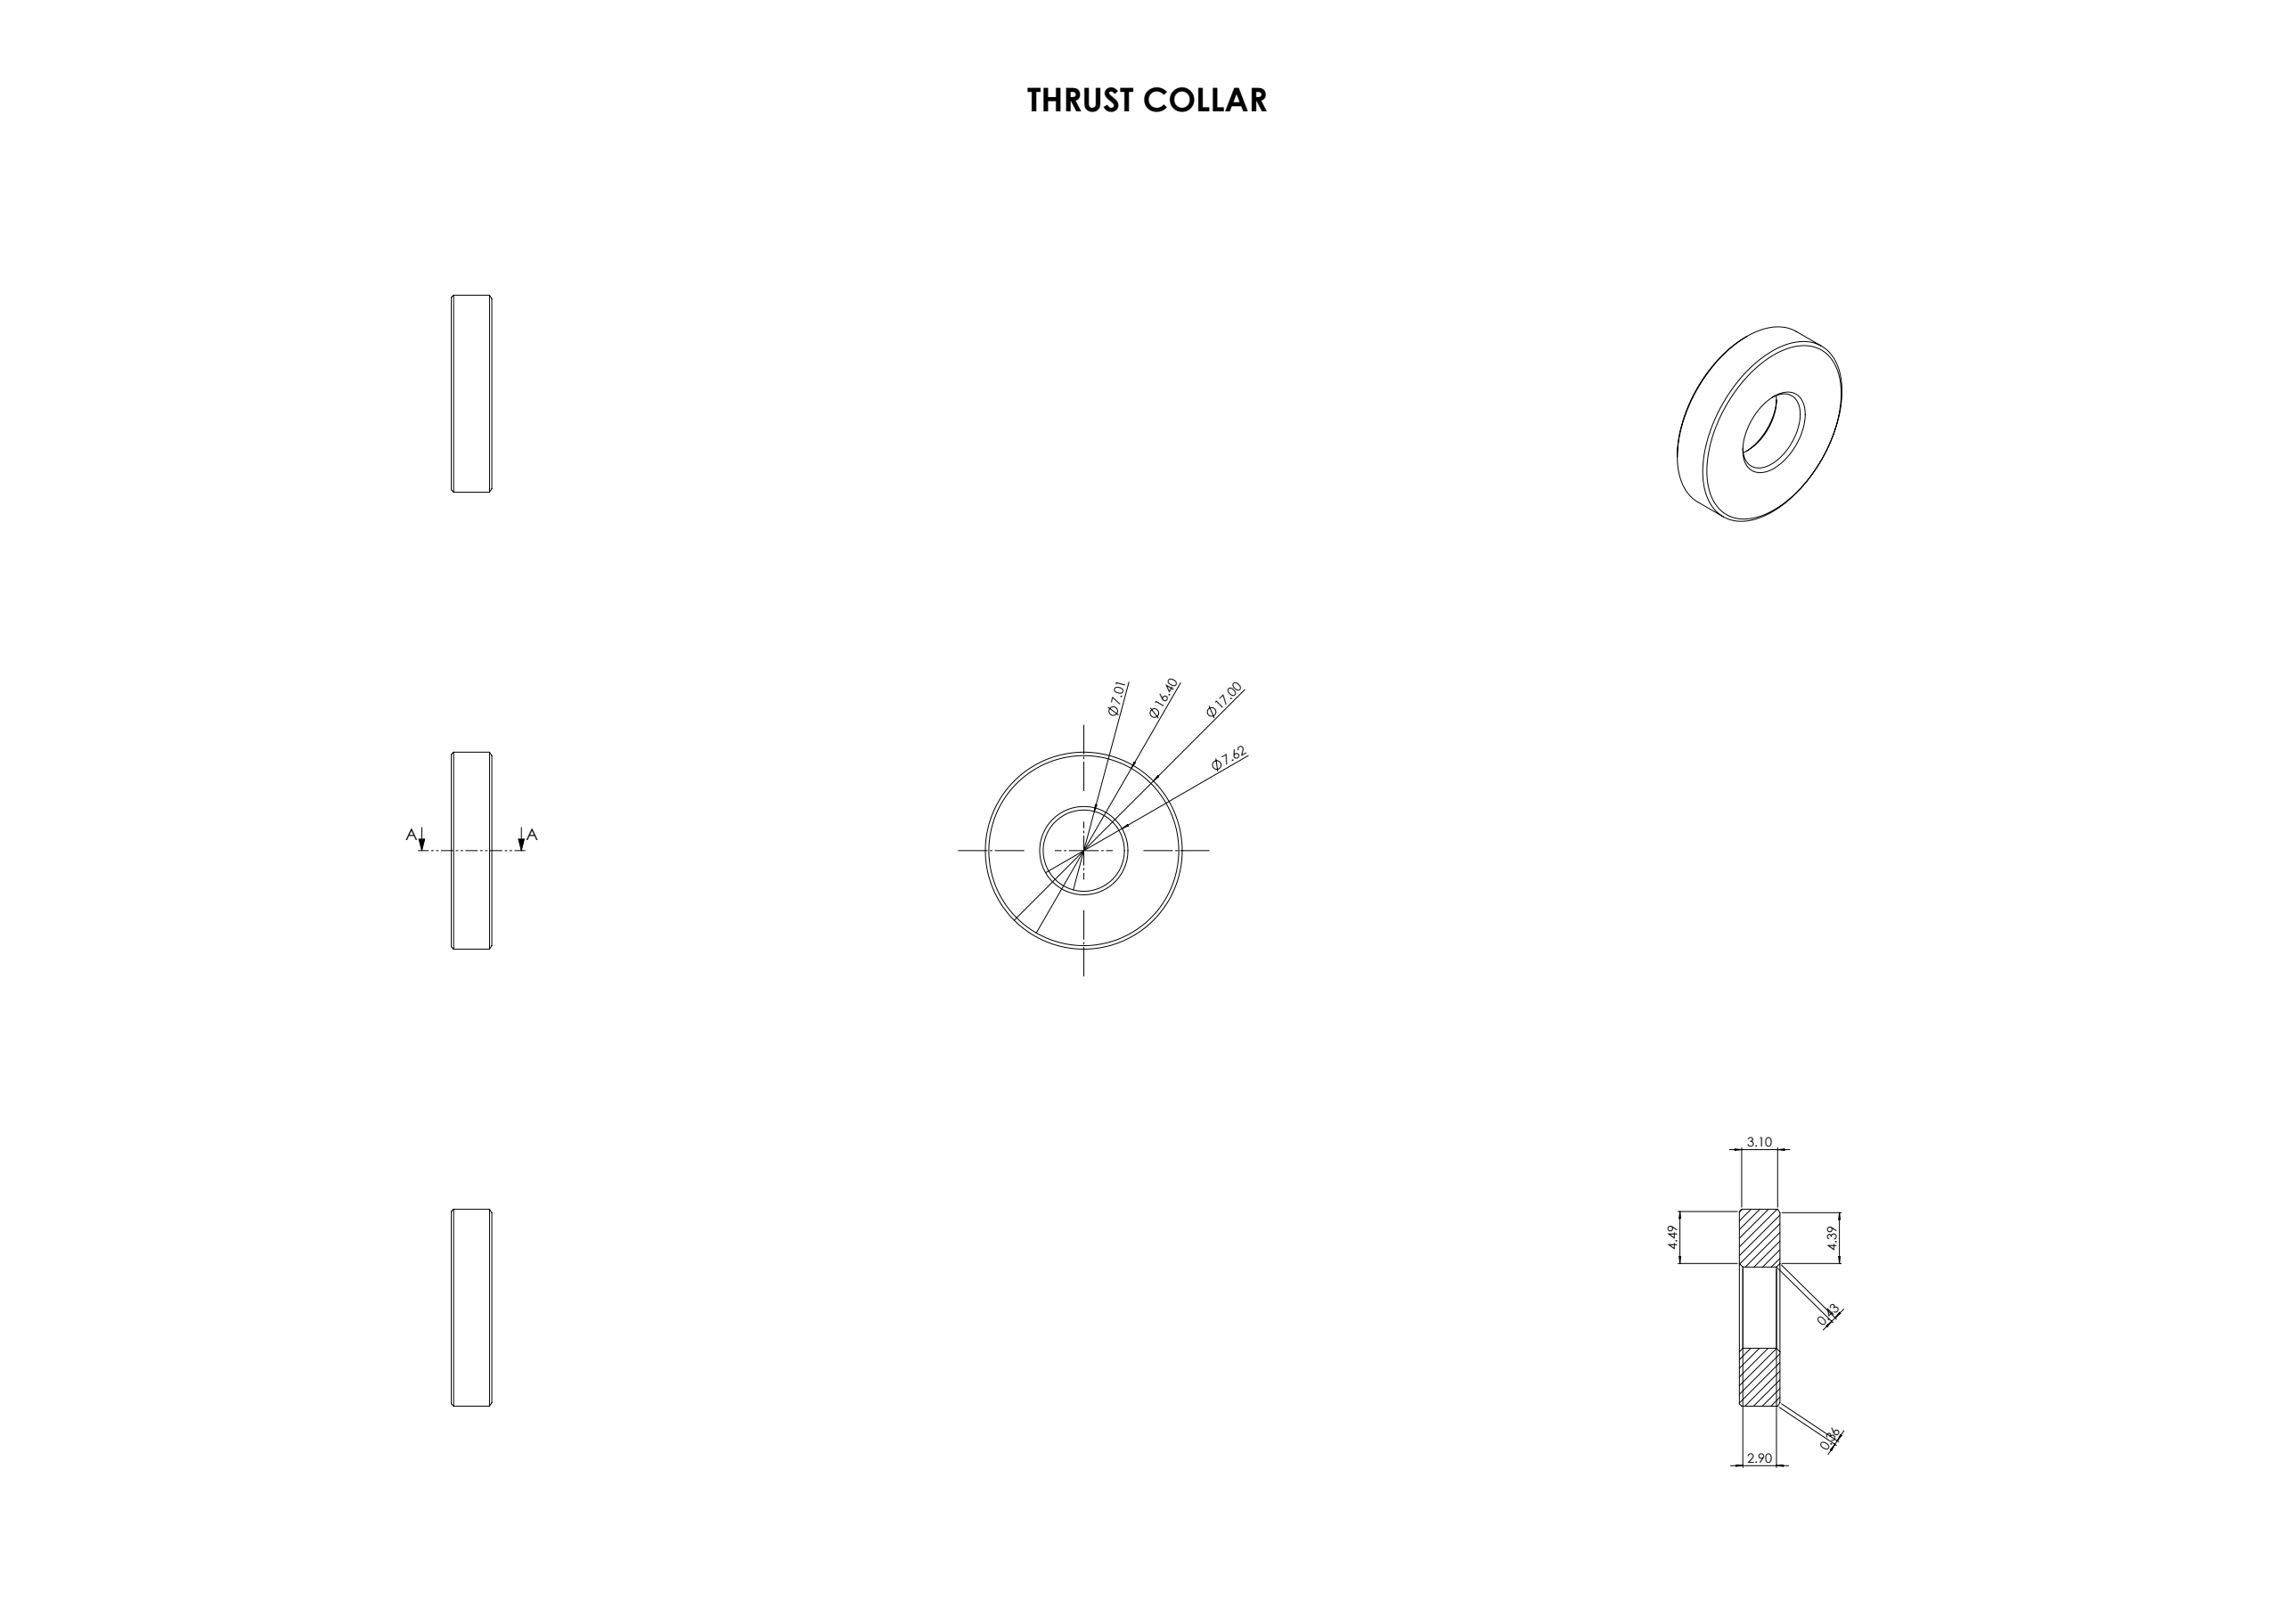
ISO-10303-21;
HEADER;
/* Generated by software containing ST-Developer
 * from STEP Tools, Inc. (www.steptools.com) 
 */

FILE_DESCRIPTION(
/* description */ (''),
/* implementation_level */ '2;1');

FILE_NAME(
/* name */ '05_Thrust_Collar.step',
/* time_stamp */ '2026-10-25T01:10:36-07:00',
/* author */ (''),
/* organization */ (''),
/* preprocessor_version */ 'ST-DEVELOPER v20.2',
/* originating_system */ 'Autodesk Translation Framework v15.15.0.0',
/* authorisation */ '');

FILE_SCHEMA (('AUTOMOTIVE_DESIGN { 1 0 10303 214 3 1 1 }'));
ENDSEC;

DATA;
#10=MECHANICAL_DESIGN_GEOMETRIC_PRESENTATION_REPRESENTATION('',(#1297),#60365);
#69=SHAPE_REPRESENTATION_RELATIONSHIP('SRR','None',#60409,#79);
#79=ADVANCED_BREP_SHAPE_REPRESENTATION('',(#89),#60357);
#89=MANIFOLD_SOLID_BREP('Body1',#18299);
#206=FACE_BOUND('',#2619,.T.);
#207=FACE_BOUND('',#2624,.T.);
#401=PLANE('',#18929);
#402=PLANE('',#18937);
#902=CONICAL_SURFACE('',#18922,8.4,0.785398163397446);
#903=CONICAL_SURFACE('',#18927,8.35,0.982793723247329);
#904=CONICAL_SURFACE('',#18931,3.6575,0.7936624380571);
#905=CONICAL_SURFACE('',#18935,3.6575,0.7936624380571);
#1297=STYLED_ITEM('',(#60541),#89);
#1642=FACE_OUTER_BOUND('',#2615,.T.);
#1643=FACE_OUTER_BOUND('',#2616,.T.);
#1644=FACE_OUTER_BOUND('',#2617,.T.);
#1645=FACE_OUTER_BOUND('',#2618,.T.);
#1646=FACE_OUTER_BOUND('',#2620,.T.);
#1647=FACE_OUTER_BOUND('',#2621,.T.);
#1648=FACE_OUTER_BOUND('',#2622,.T.);
#1649=FACE_OUTER_BOUND('',#2623,.T.);
#2615=EDGE_LOOP('',(#13723,#13724,#13725,#13726));
#2616=EDGE_LOOP('',(#13727,#13728,#13729,#13730));
#2617=EDGE_LOOP('',(#13731,#13732,#13733,#13734));
#2618=EDGE_LOOP('',(#13735));
#2619=EDGE_LOOP('',(#13736));
#2620=EDGE_LOOP('',(#13737,#13738,#13739,#13740));
#2621=EDGE_LOOP('',(#13741,#13742,#13743,#13744));
#2622=EDGE_LOOP('',(#13745,#13746,#13747,#13748));
#2623=EDGE_LOOP('',(#13749));
#2624=EDGE_LOOP('',(#13750));
#3509=CIRCLE('',#18923,8.5);
#3510=CIRCLE('',#18924,8.3);
#3511=CIRCLE('',#18926,8.5);
#3512=CIRCLE('',#18928,8.2);
#3513=CIRCLE('',#18930,3.81);
#3514=CIRCLE('',#18932,3.505);
#3515=CIRCLE('',#18934,3.505);
#3516=CIRCLE('',#18936,3.81);
#4780=LINE('',#43732,#6192);
#4781=LINE('',#43737,#6193);
#4782=LINE('',#43741,#6194);
#4783=LINE('',#43747,#6195);
#4784=LINE('',#43751,#6196);
#4785=LINE('',#43755,#6197);
#6192=VECTOR('',#20970,8.4);
#6193=VECTOR('',#20977,8.5);
#6194=VECTOR('',#20982,8.35);
#6195=VECTOR('',#20989,3.6575);
#6196=VECTOR('',#20994,3.505);
#6197=VECTOR('',#20999,3.6575);
#7954=VERTEX_POINT('',#43729);
#7955=VERTEX_POINT('',#43731);
#7956=VERTEX_POINT('',#43735);
#7957=VERTEX_POINT('',#43739);
#7958=VERTEX_POINT('',#43743);
#7959=VERTEX_POINT('',#43746);
#7960=VERTEX_POINT('',#43750);
#7961=VERTEX_POINT('',#43754);
#10069=EDGE_CURVE('',#7954,#7954,#3509,.T.);
#10070=EDGE_CURVE('',#7954,#7955,#4780,.T.);
#10071=EDGE_CURVE('',#7955,#7955,#3510,.T.);
#10072=EDGE_CURVE('',#7956,#7956,#3511,.T.);
#10073=EDGE_CURVE('',#7956,#7954,#4781,.T.);
#10074=EDGE_CURVE('',#7957,#7957,#3512,.T.);
#10075=EDGE_CURVE('',#7957,#7956,#4782,.T.);
#10076=EDGE_CURVE('',#7958,#7958,#3513,.T.);
#10077=EDGE_CURVE('',#7958,#7959,#4783,.T.);
#10078=EDGE_CURVE('',#7959,#7959,#3514,.T.);
#10079=EDGE_CURVE('',#7959,#7960,#4784,.T.);
#10080=EDGE_CURVE('',#7960,#7960,#3515,.T.);
#10081=EDGE_CURVE('',#7960,#7961,#4785,.T.);
#10082=EDGE_CURVE('',#7961,#7961,#3516,.T.);
#13723=ORIENTED_EDGE('',*,*,#10069,.F.);
#13724=ORIENTED_EDGE('',*,*,#10070,.T.);
#13725=ORIENTED_EDGE('',*,*,#10071,.T.);
#13726=ORIENTED_EDGE('',*,*,#10070,.F.);
#13727=ORIENTED_EDGE('',*,*,#10072,.F.);
#13728=ORIENTED_EDGE('',*,*,#10073,.T.);
#13729=ORIENTED_EDGE('',*,*,#10069,.T.);
#13730=ORIENTED_EDGE('',*,*,#10073,.F.);
#13731=ORIENTED_EDGE('',*,*,#10074,.F.);
#13732=ORIENTED_EDGE('',*,*,#10075,.T.);
#13733=ORIENTED_EDGE('',*,*,#10072,.T.);
#13734=ORIENTED_EDGE('',*,*,#10075,.F.);
#13735=ORIENTED_EDGE('',*,*,#10074,.T.);
#13736=ORIENTED_EDGE('',*,*,#10076,.F.);
#13737=ORIENTED_EDGE('',*,*,#10076,.T.);
#13738=ORIENTED_EDGE('',*,*,#10077,.T.);
#13739=ORIENTED_EDGE('',*,*,#10078,.F.);
#13740=ORIENTED_EDGE('',*,*,#10077,.F.);
#13741=ORIENTED_EDGE('',*,*,#10078,.T.);
#13742=ORIENTED_EDGE('',*,*,#10079,.T.);
#13743=ORIENTED_EDGE('',*,*,#10080,.F.);
#13744=ORIENTED_EDGE('',*,*,#10079,.F.);
#13745=ORIENTED_EDGE('',*,*,#10080,.T.);
#13746=ORIENTED_EDGE('',*,*,#10081,.T.);
#13747=ORIENTED_EDGE('',*,*,#10082,.F.);
#13748=ORIENTED_EDGE('',*,*,#10081,.F.);
#13749=ORIENTED_EDGE('',*,*,#10071,.F.);
#13750=ORIENTED_EDGE('',*,*,#10082,.T.);
#17294=CYLINDRICAL_SURFACE('',#18925,8.5);
#17295=CYLINDRICAL_SURFACE('',#18933,3.505);
#17670=ADVANCED_FACE('',(#1642),#902,.T.);
#17671=ADVANCED_FACE('',(#1643),#17294,.T.);
#17672=ADVANCED_FACE('',(#1644),#903,.T.);
#17673=ADVANCED_FACE('',(#1645,#206),#401,.T.);
#17674=ADVANCED_FACE('',(#1646),#904,.F.);
#17675=ADVANCED_FACE('',(#1647),#17295,.F.);
#17676=ADVANCED_FACE('',(#1648),#905,.F.);
#17677=ADVANCED_FACE('',(#1649,#207),#402,.T.);
#18299=CLOSED_SHELL('',(#17670,#17671,#17672,#17673,#17674,#17675,#17676,
#17677));
#18921=AXIS2_PLACEMENT_3D('',#43727,#20964,#20965);
#18922=AXIS2_PLACEMENT_3D('',#43728,#20966,#20967);
#18923=AXIS2_PLACEMENT_3D('',#43730,#20968,#20969);
#18924=AXIS2_PLACEMENT_3D('',#43733,#20971,#20972);
#18925=AXIS2_PLACEMENT_3D('',#43734,#20973,#20974);
#18926=AXIS2_PLACEMENT_3D('',#43736,#20975,#20976);
#18927=AXIS2_PLACEMENT_3D('',#43738,#20978,#20979);
#18928=AXIS2_PLACEMENT_3D('',#43740,#20980,#20981);
#18929=AXIS2_PLACEMENT_3D('',#43742,#20983,#20984);
#18930=AXIS2_PLACEMENT_3D('',#43744,#20985,#20986);
#18931=AXIS2_PLACEMENT_3D('',#43745,#20987,#20988);
#18932=AXIS2_PLACEMENT_3D('',#43748,#20990,#20991);
#18933=AXIS2_PLACEMENT_3D('',#43749,#20992,#20993);
#18934=AXIS2_PLACEMENT_3D('',#43752,#20995,#20996);
#18935=AXIS2_PLACEMENT_3D('',#43753,#20997,#20998);
#18936=AXIS2_PLACEMENT_3D('',#43756,#21000,#21001);
#18937=AXIS2_PLACEMENT_3D('',#43757,#21002,#21003);
#20964=DIRECTION('axis',(0.,0.,1.));
#20965=DIRECTION('refdir',(1.,0.,0.));
#20966=DIRECTION('center_axis',(1.,0.,0.));
#20967=DIRECTION('ref_axis',(0.,1.,0.));
#20968=DIRECTION('center_axis',(1.,0.,0.));
#20969=DIRECTION('ref_axis',(0.,0.,-1.));
#20970=DIRECTION('',(-0.707106781186549,0.707106781186546,8.65956056235491E-17));
#20971=DIRECTION('center_axis',(1.,0.,0.));
#20972=DIRECTION('ref_axis',(0.,0.,-1.));
#20973=DIRECTION('center_axis',(1.,0.,0.));
#20974=DIRECTION('ref_axis',(0.,1.,0.));
#20975=DIRECTION('center_axis',(1.,0.,0.));
#20976=DIRECTION('ref_axis',(0.,0.,-1.));
#20977=DIRECTION('',(-1.,0.,0.));
#20978=DIRECTION('center_axis',(-1.,0.,0.));
#20979=DIRECTION('ref_axis',(0.,1.,0.));
#20980=DIRECTION('center_axis',(1.,0.,0.));
#20981=DIRECTION('ref_axis',(0.,0.,-1.));
#20982=DIRECTION('',(-0.554700196225229,-0.832050294337844,-1.01896772969045E-16));
#20983=DIRECTION('center_axis',(1.,0.,0.));
#20984=DIRECTION('ref_axis',(0.,0.,-1.));
#20985=DIRECTION('center_axis',(1.,0.,0.));
#20986=DIRECTION('ref_axis',(0.,0.,-1.));
#20987=DIRECTION('center_axis',(1.,0.,0.));
#20988=DIRECTION('ref_axis',(0.,1.,0.));
#20989=DIRECTION('',(-0.701238976116887,0.712926292385503,8.73082901997897E-17));
#20990=DIRECTION('center_axis',(1.,0.,0.));
#20991=DIRECTION('ref_axis',(0.,0.,-1.));
#20992=DIRECTION('center_axis',(1.,0.,0.));
#20993=DIRECTION('ref_axis',(0.,1.,0.));
#20994=DIRECTION('',(-1.,0.,0.));
#20995=DIRECTION('center_axis',(1.,0.,0.));
#20996=DIRECTION('ref_axis',(0.,0.,-1.));
#20997=DIRECTION('center_axis',(-1.,0.,0.));
#20998=DIRECTION('ref_axis',(0.,1.,0.));
#20999=DIRECTION('',(-0.701238976116887,-0.712926292385503,-8.73082901997896E-17));
#21000=DIRECTION('center_axis',(1.,0.,0.));
#21001=DIRECTION('ref_axis',(0.,0.,-1.));
#21002=DIRECTION('center_axis',(-1.,0.,0.));
#21003=DIRECTION('ref_axis',(0.,0.,1.));
#43727=CARTESIAN_POINT('',(0.,0.,0.));
#43728=CARTESIAN_POINT('Origin',(0.1,0.,0.));
#43729=CARTESIAN_POINT('',(0.2,-8.5,-1.04094977927525E-15));
#43730=CARTESIAN_POINT('Origin',(0.2,0.,0.));
#43731=CARTESIAN_POINT('',(-3.98986399474666E-16,-8.3,-1.0164568432923E-15));
#43732=CARTESIAN_POINT('',(0.1,-8.4,-1.02870331128378E-15));
#43733=CARTESIAN_POINT('Origin',(0.,0.,0.));
#43734=CARTESIAN_POINT('Origin',(1.75,0.,0.));
#43735=CARTESIAN_POINT('',(3.3,-8.5,-1.04094977927525E-15));
#43736=CARTESIAN_POINT('Origin',(3.3,0.,0.));
#43737=CARTESIAN_POINT('',(1.75,-8.5,-1.04094977927525E-15));
#43738=CARTESIAN_POINT('Origin',(3.4,0.,0.));
#43739=CARTESIAN_POINT('',(3.5,-8.2,-1.00421037530083E-15));
#43740=CARTESIAN_POINT('Origin',(3.5,0.,0.));
#43741=CARTESIAN_POINT('',(3.4,-8.35,-1.02258007728804E-15));
#43742=CARTESIAN_POINT('Origin',(3.5,3.81,0.));
#43743=CARTESIAN_POINT('',(3.5,-3.81,-4.66590430475142E-16));
#43744=CARTESIAN_POINT('Origin',(3.5,0.,0.));
#43745=CARTESIAN_POINT('Origin',(3.35,0.,0.));
#43746=CARTESIAN_POINT('',(3.2,-3.505,-4.29238703101147E-16));
#43747=CARTESIAN_POINT('',(3.35,-3.6575,-4.47914566788144E-16));
#43748=CARTESIAN_POINT('Origin',(3.2,0.,0.));
#43749=CARTESIAN_POINT('Origin',(1.75,0.,0.));
#43750=CARTESIAN_POINT('',(0.3,-3.505,-4.29238703101147E-16));
#43751=CARTESIAN_POINT('',(1.75,-3.505,-4.29238703101147E-16));
#43752=CARTESIAN_POINT('Origin',(0.3,0.,0.));
#43753=CARTESIAN_POINT('Origin',(0.15,0.,0.));
#43754=CARTESIAN_POINT('',(1.21430643318376E-16,-3.81,-4.66590430475142E-16));
#43755=CARTESIAN_POINT('',(0.15,-3.6575,-4.47914566788144E-16));
#43756=CARTESIAN_POINT('Origin',(0.,0.,0.));
#43757=CARTESIAN_POINT('Origin',(0.,8.3,0.));
#60345=UNCERTAINTY_MEASURE_WITH_UNIT(LENGTH_MEASURE(0.01),#60366,
'DISTANCE_ACCURACY_VALUE',
'Maximum model space distance between geometric entities at asserted c
onnectivities');
#60353=UNCERTAINTY_MEASURE_WITH_UNIT(LENGTH_MEASURE(0.01),#60366,
'DISTANCE_ACCURACY_VALUE',
'Maximum model space distance between geometric entities at asserted c
onnectivities');
#60357=(
GEOMETRIC_REPRESENTATION_CONTEXT(3)
GLOBAL_UNCERTAINTY_ASSIGNED_CONTEXT((#60345))
GLOBAL_UNIT_ASSIGNED_CONTEXT((#60366,#60368,#60369))
REPRESENTATION_CONTEXT('','3D')
);
#60365=(
GEOMETRIC_REPRESENTATION_CONTEXT(3)
GLOBAL_UNCERTAINTY_ASSIGNED_CONTEXT((#60353))
GLOBAL_UNIT_ASSIGNED_CONTEXT((#60366,#60368,#60369))
REPRESENTATION_CONTEXT('','3D')
);
#60366=(
LENGTH_UNIT()
NAMED_UNIT(*)
SI_UNIT(.MILLI.,.METRE.)
);
#60368=(
NAMED_UNIT(*)
PLANE_ANGLE_UNIT()
SI_UNIT($,.RADIAN.)
);
#60369=(
NAMED_UNIT(*)
SI_UNIT($,.STERADIAN.)
SOLID_ANGLE_UNIT()
);
#60373=SHAPE_DEFINITION_REPRESENTATION(#60384,#60409);
#60384=PRODUCT_DEFINITION_SHAPE('',$,#60421);
#60409=SHAPE_REPRESENTATION('',(#18921),#60357);
#60417=PRODUCT_DEFINITION_CONTEXT('part definition',#60452,'design');
#60421=PRODUCT_DEFINITION('2026-10-25-00-06-30-524','05_Thrust_Collar',
#60432,#60417);
#60432=PRODUCT_DEFINITION_FORMATION('',$,#60457);
#60452=APPLICATION_CONTEXT(
'Core Data for Automotive Mechanical Design Process');
#60453=PRODUCT_CONTEXT('part definition',#60452,'mechanical');
#60457=PRODUCT('2026-10-25-00-06-30-524','05_Thrust_Collar',$,(#60453));
#60535=COLOUR_RGB('Off White',0.89,0.88,0.83);
#60536=FILL_AREA_STYLE_COLOUR('',#60535);
#60537=FILL_AREA_STYLE('',(#60536));
#60538=SURFACE_STYLE_FILL_AREA(#60537);
#60539=SURFACE_SIDE_STYLE('',(#60538));
#60540=SURFACE_STYLE_USAGE(.BOTH.,#60539);
#60541=PRESENTATION_STYLE_ASSIGNMENT((#60540));
ENDSEC;
END-ISO-10303-21;
